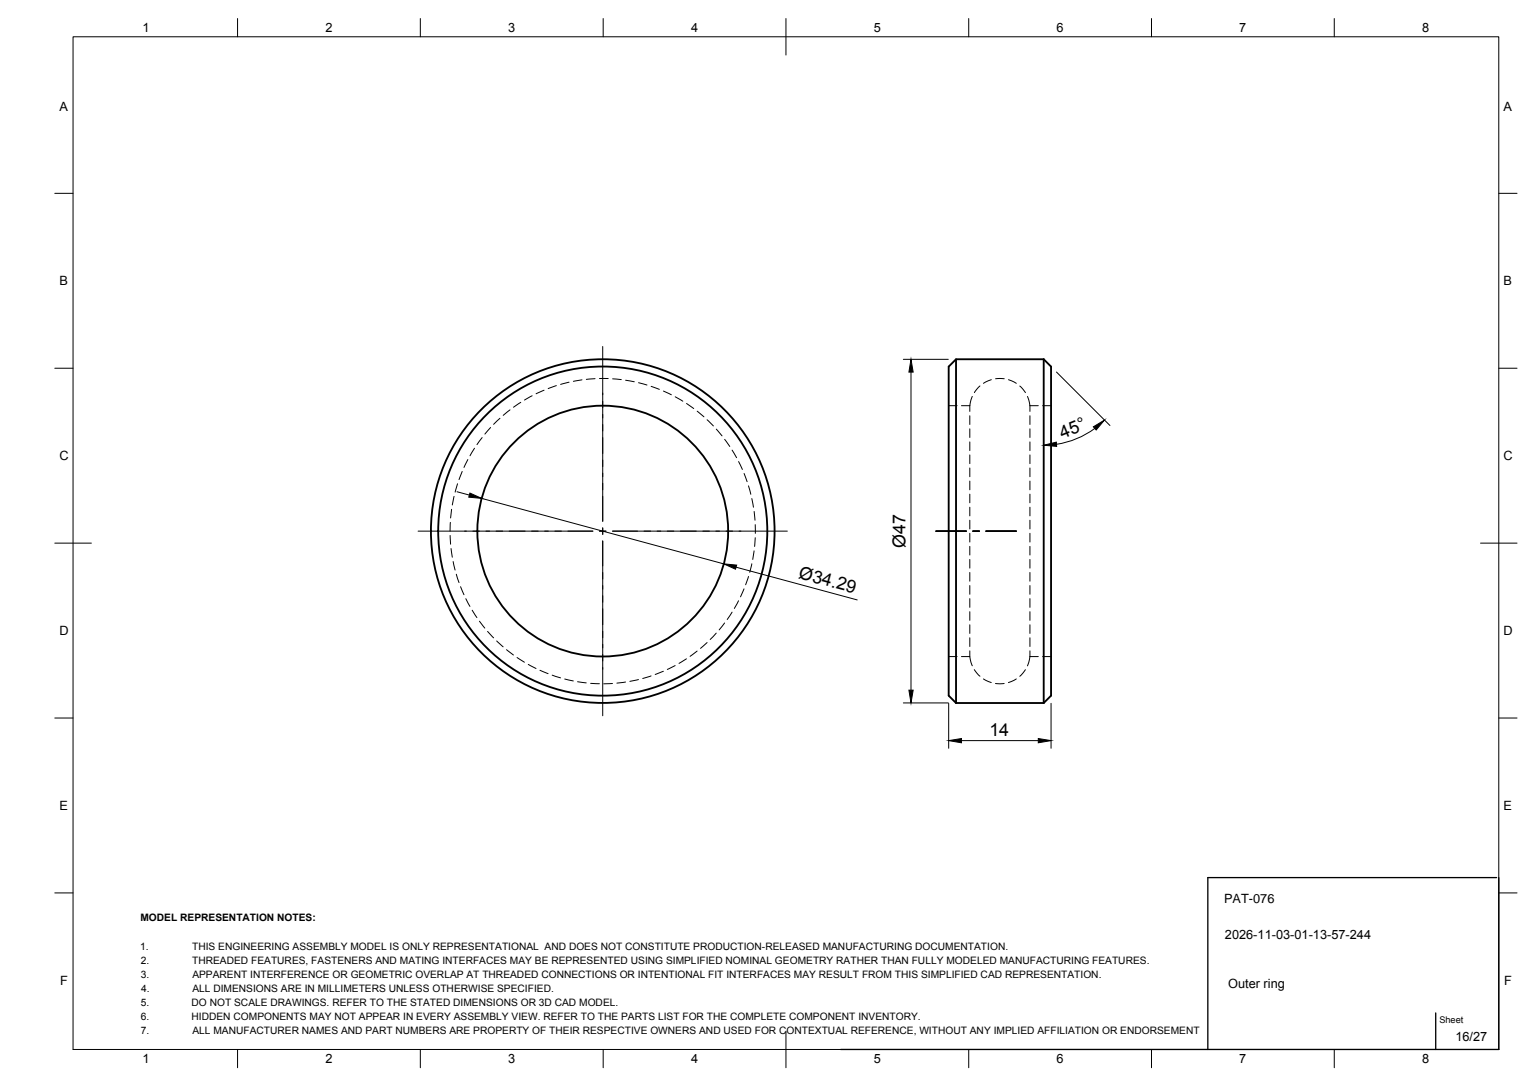
ISO-10303-21;
HEADER;
/* Generated by software containing ST-Developer
 * from STEP Tools, Inc. (www.steptools.com) 
 */

FILE_DESCRIPTION(
/* description */ ('Overhung pulley bearing cartridge'),
/* implementation_level */ '2;1');

FILE_NAME(
/* name */ 'Outer ring.step',
/* time_stamp */ '2026-10-28T03:22:33-07:00',
/* author */ (''),
/* organization */ (''),
/* preprocessor_version */ 'ST-DEVELOPER v20.2',
/* originating_system */ 'Autodesk Translation Framework v15.17.0.0',
/* authorisation */ '');

FILE_SCHEMA (('AUTOMOTIVE_DESIGN { 1 0 10303 214 3 1 1 }'));
ENDSEC;

DATA;
#10=MECHANICAL_DESIGN_GEOMETRIC_PRESENTATION_REPRESENTATION('',(#292),#10963);
#225=CONICAL_SURFACE('',#6144,2.3,0.785398163397449);
#226=CONICAL_SURFACE('',#6148,2.3,0.785398163397449);
#238=TOROIDAL_SURFACE('',#6133,1.675,0.412776);
#248=SHAPE_REPRESENTATION_RELATIONSHIP('SRR','None',#11069,#270);
#270=ADVANCED_BREP_SHAPE_REPRESENTATION('',(#322),#10949);
#292=STYLED_ITEM('',(#11253),#322);
#322=MANIFOLD_SOLID_BREP('Body1',#5659);
#398=FACE_BOUND('',#1068,.T.);
#399=FACE_BOUND('',#1073,.T.);
#493=PLANE('',#6141);
#494=PLANE('',#6150);
#679=FACE_OUTER_BOUND('',#1065,.T.);
#680=FACE_OUTER_BOUND('',#1066,.T.);
#681=FACE_OUTER_BOUND('',#1067,.T.);
#682=FACE_OUTER_BOUND('',#1069,.T.);
#683=FACE_OUTER_BOUND('',#1070,.T.);
#684=FACE_OUTER_BOUND('',#1071,.T.);
#685=FACE_OUTER_BOUND('',#1072,.T.);
#686=FACE_OUTER_BOUND('',#1074,.T.);
#1065=EDGE_LOOP('',(#4067,#4068,#4069,#4070,#4071,#4072));
#1066=EDGE_LOOP('',(#4073,#4074,#4075,#4076,#4077));
#1067=EDGE_LOOP('',(#4078));
#1068=EDGE_LOOP('',(#4079));
#1069=EDGE_LOOP('',(#4080,#4081,#4082,#4083));
#1070=EDGE_LOOP('',(#4084,#4085,#4086,#4087));
#1071=EDGE_LOOP('',(#4088,#4089,#4090,#4091));
#1072=EDGE_LOOP('',(#4092));
#1073=EDGE_LOOP('',(#4093));
#1074=EDGE_LOOP('',(#4094,#4095,#4096,#4097,#4098));
#1442=LINE('',#9027,#1784);
#1443=LINE('',#9036,#1785);
#1444=LINE('',#9040,#1786);
#1445=LINE('',#9044,#1787);
#1446=LINE('',#9047,#1788);
#1784=VECTOR('',#7234,1.71469);
#1785=VECTOR('',#7245,2.3);
#1786=VECTOR('',#7250,2.35);
#1787=VECTOR('',#7255,2.3);
#1788=VECTOR('',#7260,1.71469);
#2105=CIRCLE('',#6134,1.71469);
#2106=CIRCLE('',#6135,1.71469);
#2107=CIRCLE('',#6136,0.412776);
#2108=CIRCLE('',#6137,1.71469);
#2109=CIRCLE('',#6138,1.71469);
#2110=CIRCLE('',#6140,1.71469);
#2111=CIRCLE('',#6142,2.25);
#2112=CIRCLE('',#6143,1.71469);
#2113=CIRCLE('',#6145,2.35);
#2114=CIRCLE('',#6147,2.35);
#2115=CIRCLE('',#6149,2.25);
#2519=VERTEX_POINT('',#9015);
#2520=VERTEX_POINT('',#9016);
#2521=VERTEX_POINT('',#9019);
#2522=VERTEX_POINT('',#9021);
#2523=VERTEX_POINT('',#9025);
#2524=VERTEX_POINT('',#9029);
#2525=VERTEX_POINT('',#9031);
#2526=VERTEX_POINT('',#9034);
#2527=VERTEX_POINT('',#9038);
#2528=VERTEX_POINT('',#9042);
#3103=EDGE_CURVE('',#2519,#2520,#2105,.T.);
#3104=EDGE_CURVE('',#2520,#2519,#2106,.T.);
#3105=EDGE_CURVE('',#2520,#2521,#2107,.T.);
#3106=EDGE_CURVE('',#2522,#2521,#2108,.T.);
#3107=EDGE_CURVE('',#2521,#2522,#2109,.T.);
#3108=EDGE_CURVE('',#2523,#2523,#2110,.T.);
#3109=EDGE_CURVE('',#2523,#2522,#1442,.T.);
#3110=EDGE_CURVE('',#2524,#2524,#2111,.T.);
#3111=EDGE_CURVE('',#2525,#2525,#2112,.T.);
#3112=EDGE_CURVE('',#2526,#2526,#2113,.T.);
#3113=EDGE_CURVE('',#2526,#2524,#1443,.T.);
#3114=EDGE_CURVE('',#2527,#2527,#2114,.T.);
#3115=EDGE_CURVE('',#2527,#2526,#1444,.T.);
#3116=EDGE_CURVE('',#2528,#2528,#2115,.T.);
#3117=EDGE_CURVE('',#2528,#2527,#1445,.T.);
#3118=EDGE_CURVE('',#2519,#2525,#1446,.T.);
#4067=ORIENTED_EDGE('',*,*,#3103,.F.);
#4068=ORIENTED_EDGE('',*,*,#3104,.F.);
#4069=ORIENTED_EDGE('',*,*,#3105,.T.);
#4070=ORIENTED_EDGE('',*,*,#3106,.F.);
#4071=ORIENTED_EDGE('',*,*,#3107,.F.);
#4072=ORIENTED_EDGE('',*,*,#3105,.F.);
#4073=ORIENTED_EDGE('',*,*,#3108,.T.);
#4074=ORIENTED_EDGE('',*,*,#3109,.T.);
#4075=ORIENTED_EDGE('',*,*,#3106,.T.);
#4076=ORIENTED_EDGE('',*,*,#3107,.T.);
#4077=ORIENTED_EDGE('',*,*,#3109,.F.);
#4078=ORIENTED_EDGE('',*,*,#3110,.F.);
#4079=ORIENTED_EDGE('',*,*,#3111,.T.);
#4080=ORIENTED_EDGE('',*,*,#3112,.F.);
#4081=ORIENTED_EDGE('',*,*,#3113,.T.);
#4082=ORIENTED_EDGE('',*,*,#3110,.T.);
#4083=ORIENTED_EDGE('',*,*,#3113,.F.);
#4084=ORIENTED_EDGE('',*,*,#3114,.F.);
#4085=ORIENTED_EDGE('',*,*,#3115,.T.);
#4086=ORIENTED_EDGE('',*,*,#3112,.T.);
#4087=ORIENTED_EDGE('',*,*,#3115,.F.);
#4088=ORIENTED_EDGE('',*,*,#3116,.F.);
#4089=ORIENTED_EDGE('',*,*,#3117,.T.);
#4090=ORIENTED_EDGE('',*,*,#3114,.T.);
#4091=ORIENTED_EDGE('',*,*,#3117,.F.);
#4092=ORIENTED_EDGE('',*,*,#3116,.T.);
#4093=ORIENTED_EDGE('',*,*,#3108,.F.);
#4094=ORIENTED_EDGE('',*,*,#3103,.T.);
#4095=ORIENTED_EDGE('',*,*,#3104,.T.);
#4096=ORIENTED_EDGE('',*,*,#3118,.T.);
#4097=ORIENTED_EDGE('',*,*,#3111,.F.);
#4098=ORIENTED_EDGE('',*,*,#3118,.F.);
#5207=CYLINDRICAL_SURFACE('',#6139,1.71469);
#5208=CYLINDRICAL_SURFACE('',#6146,2.35);
#5209=CYLINDRICAL_SURFACE('',#6151,1.71469);
#5423=ADVANCED_FACE('',(#679),#238,.F.);
#5424=ADVANCED_FACE('',(#680),#5207,.F.);
#5425=ADVANCED_FACE('',(#681,#398),#493,.T.);
#5426=ADVANCED_FACE('',(#682),#225,.T.);
#5427=ADVANCED_FACE('',(#683),#5208,.T.);
#5428=ADVANCED_FACE('',(#684),#226,.T.);
#5429=ADVANCED_FACE('',(#685,#399),#494,.T.);
#5430=ADVANCED_FACE('',(#686),#5209,.F.);
#5659=CLOSED_SHELL('',(#5423,#5424,#5425,#5426,#5427,#5428,#5429,#5430));
#6132=AXIS2_PLACEMENT_3D('',#9013,#7216,#7217);
#6133=AXIS2_PLACEMENT_3D('',#9014,#7218,#7219);
#6134=AXIS2_PLACEMENT_3D('',#9017,#7220,#7221);
#6135=AXIS2_PLACEMENT_3D('',#9018,#7222,#7223);
#6136=AXIS2_PLACEMENT_3D('',#9020,#7224,#7225);
#6137=AXIS2_PLACEMENT_3D('',#9022,#7226,#7227);
#6138=AXIS2_PLACEMENT_3D('',#9023,#7228,#7229);
#6139=AXIS2_PLACEMENT_3D('',#9024,#7230,#7231);
#6140=AXIS2_PLACEMENT_3D('',#9026,#7232,#7233);
#6141=AXIS2_PLACEMENT_3D('',#9028,#7235,#7236);
#6142=AXIS2_PLACEMENT_3D('',#9030,#7237,#7238);
#6143=AXIS2_PLACEMENT_3D('',#9032,#7239,#7240);
#6144=AXIS2_PLACEMENT_3D('',#9033,#7241,#7242);
#6145=AXIS2_PLACEMENT_3D('',#9035,#7243,#7244);
#6146=AXIS2_PLACEMENT_3D('',#9037,#7246,#7247);
#6147=AXIS2_PLACEMENT_3D('',#9039,#7248,#7249);
#6148=AXIS2_PLACEMENT_3D('',#9041,#7251,#7252);
#6149=AXIS2_PLACEMENT_3D('',#9043,#7253,#7254);
#6150=AXIS2_PLACEMENT_3D('',#9045,#7256,#7257);
#6151=AXIS2_PLACEMENT_3D('',#9046,#7258,#7259);
#7216=DIRECTION('axis',(0.,0.,1.));
#7217=DIRECTION('refdir',(1.,0.,0.));
#7218=DIRECTION('center_axis',(0.,-1.,0.));
#7219=DIRECTION('ref_axis',(0.,0.,-1.));
#7220=DIRECTION('center_axis',(0.,-1.,0.));
#7221=DIRECTION('ref_axis',(1.,0.,0.));
#7222=DIRECTION('center_axis',(0.,-1.,0.));
#7223=DIRECTION('ref_axis',(1.,0.,0.));
#7224=DIRECTION('center_axis',(1.,0.,1.22464679914735E-16));
#7225=DIRECTION('ref_axis',(-1.22464679914735E-16,0.,1.));
#7226=DIRECTION('center_axis',(0.,1.,0.));
#7227=DIRECTION('ref_axis',(1.,0.,0.));
#7228=DIRECTION('center_axis',(0.,1.,0.));
#7229=DIRECTION('ref_axis',(1.,0.,0.));
#7230=DIRECTION('center_axis',(0.,-1.,0.));
#7231=DIRECTION('ref_axis',(1.,0.,0.));
#7232=DIRECTION('center_axis',(0.,-1.,0.));
#7233=DIRECTION('ref_axis',(1.,0.,0.));
#7234=DIRECTION('',(0.,1.,0.));
#7235=DIRECTION('center_axis',(0.,1.,0.));
#7236=DIRECTION('ref_axis',(0.,0.,1.));
#7237=DIRECTION('center_axis',(0.,-1.,0.));
#7238=DIRECTION('ref_axis',(1.,0.,0.));
#7239=DIRECTION('center_axis',(0.,-1.,0.));
#7240=DIRECTION('ref_axis',(1.,0.,0.));
#7241=DIRECTION('center_axis',(0.,-1.,0.));
#7242=DIRECTION('ref_axis',(1.,0.,0.));
#7243=DIRECTION('center_axis',(0.,-1.,0.));
#7244=DIRECTION('ref_axis',(1.,0.,0.));
#7245=DIRECTION('',(0.707106781186548,0.707106781186547,8.65956056235494E-17));
#7246=DIRECTION('center_axis',(0.,-1.,0.));
#7247=DIRECTION('ref_axis',(1.,0.,0.));
#7248=DIRECTION('center_axis',(0.,-1.,0.));
#7249=DIRECTION('ref_axis',(1.,0.,0.));
#7250=DIRECTION('',(0.,1.,0.));
#7251=DIRECTION('center_axis',(0.,1.,0.));
#7252=DIRECTION('ref_axis',(1.,0.,0.));
#7253=DIRECTION('center_axis',(0.,-1.,0.));
#7254=DIRECTION('ref_axis',(1.,0.,0.));
#7255=DIRECTION('',(-0.707106781186548,0.707106781186547,-8.65956056235494E-17));
#7256=DIRECTION('center_axis',(0.,-1.,0.));
#7257=DIRECTION('ref_axis',(0.,0.,-1.));
#7258=DIRECTION('center_axis',(0.,-1.,0.));
#7259=DIRECTION('ref_axis',(1.,0.,0.));
#7260=DIRECTION('',(0.,1.,0.));
#9013=CARTESIAN_POINT('',(0.,0.,0.));
#9014=CARTESIAN_POINT('Origin',(0.,0.,0.));
#9015=CARTESIAN_POINT('',(-1.71469,0.410863395882378,-2.09988962002998E-16));
#9016=CARTESIAN_POINT('',(-2.09988962002998E-16,0.410863395882378,1.71469));
#9017=CARTESIAN_POINT('Origin',(0.,0.410863395882378,0.));
#9018=CARTESIAN_POINT('Origin',(0.,0.410863395882378,0.));
#9019=CARTESIAN_POINT('',(-2.09988962002998E-16,-0.410863395882378,1.71469));
#9020=CARTESIAN_POINT('Origin',(-2.05128338857182E-16,0.,1.675));
#9021=CARTESIAN_POINT('',(-1.71469,-0.410863395882378,2.09988962002998E-16));
#9022=CARTESIAN_POINT('Origin',(0.,-0.410863395882378,0.));
#9023=CARTESIAN_POINT('Origin',(0.,-0.410863395882378,0.));
#9024=CARTESIAN_POINT('Origin',(0.,0.,0.));
#9025=CARTESIAN_POINT('',(-1.71469,-0.7,-2.09988962002998E-16));
#9026=CARTESIAN_POINT('Origin',(0.,-0.7,0.));
#9027=CARTESIAN_POINT('',(-1.71469,0.,-2.09988962002998E-16));
#9028=CARTESIAN_POINT('Origin',(2.25,0.7,0.));
#9029=CARTESIAN_POINT('',(-2.25,0.7,-2.75545529808154E-16));
#9030=CARTESIAN_POINT('Origin',(0.,0.7,0.));
#9031=CARTESIAN_POINT('',(-1.71469,0.7,-2.09988962002998E-16));
#9032=CARTESIAN_POINT('Origin',(0.,0.7,0.));
#9033=CARTESIAN_POINT('Origin',(0.,0.65,0.));
#9034=CARTESIAN_POINT('',(-2.35,0.6,-2.87791997799628E-16));
#9035=CARTESIAN_POINT('Origin',(0.,0.6,0.));
#9036=CARTESIAN_POINT('',(-2.3,0.65,-2.81668763803891E-16));
#9037=CARTESIAN_POINT('Origin',(0.,0.,0.));
#9038=CARTESIAN_POINT('',(-2.35,-0.6,-2.87791997799628E-16));
#9039=CARTESIAN_POINT('Origin',(0.,-0.6,0.));
#9040=CARTESIAN_POINT('',(-2.35,0.,-2.87791997799628E-16));
#9041=CARTESIAN_POINT('Origin',(0.,-0.65,0.));
#9042=CARTESIAN_POINT('',(-2.25,-0.7,-2.75545529808154E-16));
#9043=CARTESIAN_POINT('Origin',(0.,-0.7,0.));
#9044=CARTESIAN_POINT('',(-2.3,-0.65,-2.81668763803891E-16));
#9045=CARTESIAN_POINT('Origin',(1.71469,-0.7,0.));
#9046=CARTESIAN_POINT('Origin',(0.,0.,0.));
#9047=CARTESIAN_POINT('',(-1.71469,0.,-2.09988962002998E-16));
#10922=UNCERTAINTY_MEASURE_WITH_UNIT(LENGTH_MEASURE(0.001),#10964,
'DISTANCE_ACCURACY_VALUE',
'Maximum model space distance between geometric entities at asserted c
onnectivities');
#10936=UNCERTAINTY_MEASURE_WITH_UNIT(LENGTH_MEASURE(0.001),#10964,
'DISTANCE_ACCURACY_VALUE',
'Maximum model space distance between geometric entities at asserted c
onnectivities');
#10949=(
GEOMETRIC_REPRESENTATION_CONTEXT(3)
GLOBAL_UNCERTAINTY_ASSIGNED_CONTEXT((#10922))
GLOBAL_UNIT_ASSIGNED_CONTEXT((#10964,#10966,#10967))
REPRESENTATION_CONTEXT('','3D')
);
#10963=(
GEOMETRIC_REPRESENTATION_CONTEXT(3)
GLOBAL_UNCERTAINTY_ASSIGNED_CONTEXT((#10936))
GLOBAL_UNIT_ASSIGNED_CONTEXT((#10964,#10966,#10967))
REPRESENTATION_CONTEXT('','3D')
);
#10964=(
LENGTH_UNIT()
NAMED_UNIT(*)
SI_UNIT(.CENTI.,.METRE.)
);
#10966=(
NAMED_UNIT(*)
PLANE_ANGLE_UNIT()
SI_UNIT($,.RADIAN.)
);
#10967=(
NAMED_UNIT(*)
SI_UNIT($,.STERADIAN.)
SOLID_ANGLE_UNIT()
);
#10980=SHAPE_DEFINITION_REPRESENTATION(#11006,#11069);
#11006=PRODUCT_DEFINITION_SHAPE('',$,#11096);
#11069=SHAPE_REPRESENTATION('',(#6132),#10949);
#11083=PRODUCT_DEFINITION_CONTEXT('part definition',#11163,'design');
#11096=PRODUCT_DEFINITION('Outer ring','Outer ring',#11122,#11083);
#11122=PRODUCT_DEFINITION_FORMATION('',$,#11177);
#11163=APPLICATION_CONTEXT(
'Core Data for Automotive Mechanical Design Process');
#11164=PRODUCT_CONTEXT('part definition',#11163,'mechanical');
#11177=PRODUCT('Outer ring','Outer ring','Outer ring',(#11164));
#11247=COLOUR_RGB('Grey',0.48,0.52,0.57);
#11248=FILL_AREA_STYLE_COLOUR('',#11247);
#11249=FILL_AREA_STYLE('',(#11248));
#11250=SURFACE_STYLE_FILL_AREA(#11249);
#11251=SURFACE_SIDE_STYLE('',(#11250));
#11252=SURFACE_STYLE_USAGE(.BOTH.,#11251);
#11253=PRESENTATION_STYLE_ASSIGNMENT((#11252));
ENDSEC;
END-ISO-10303-21;
